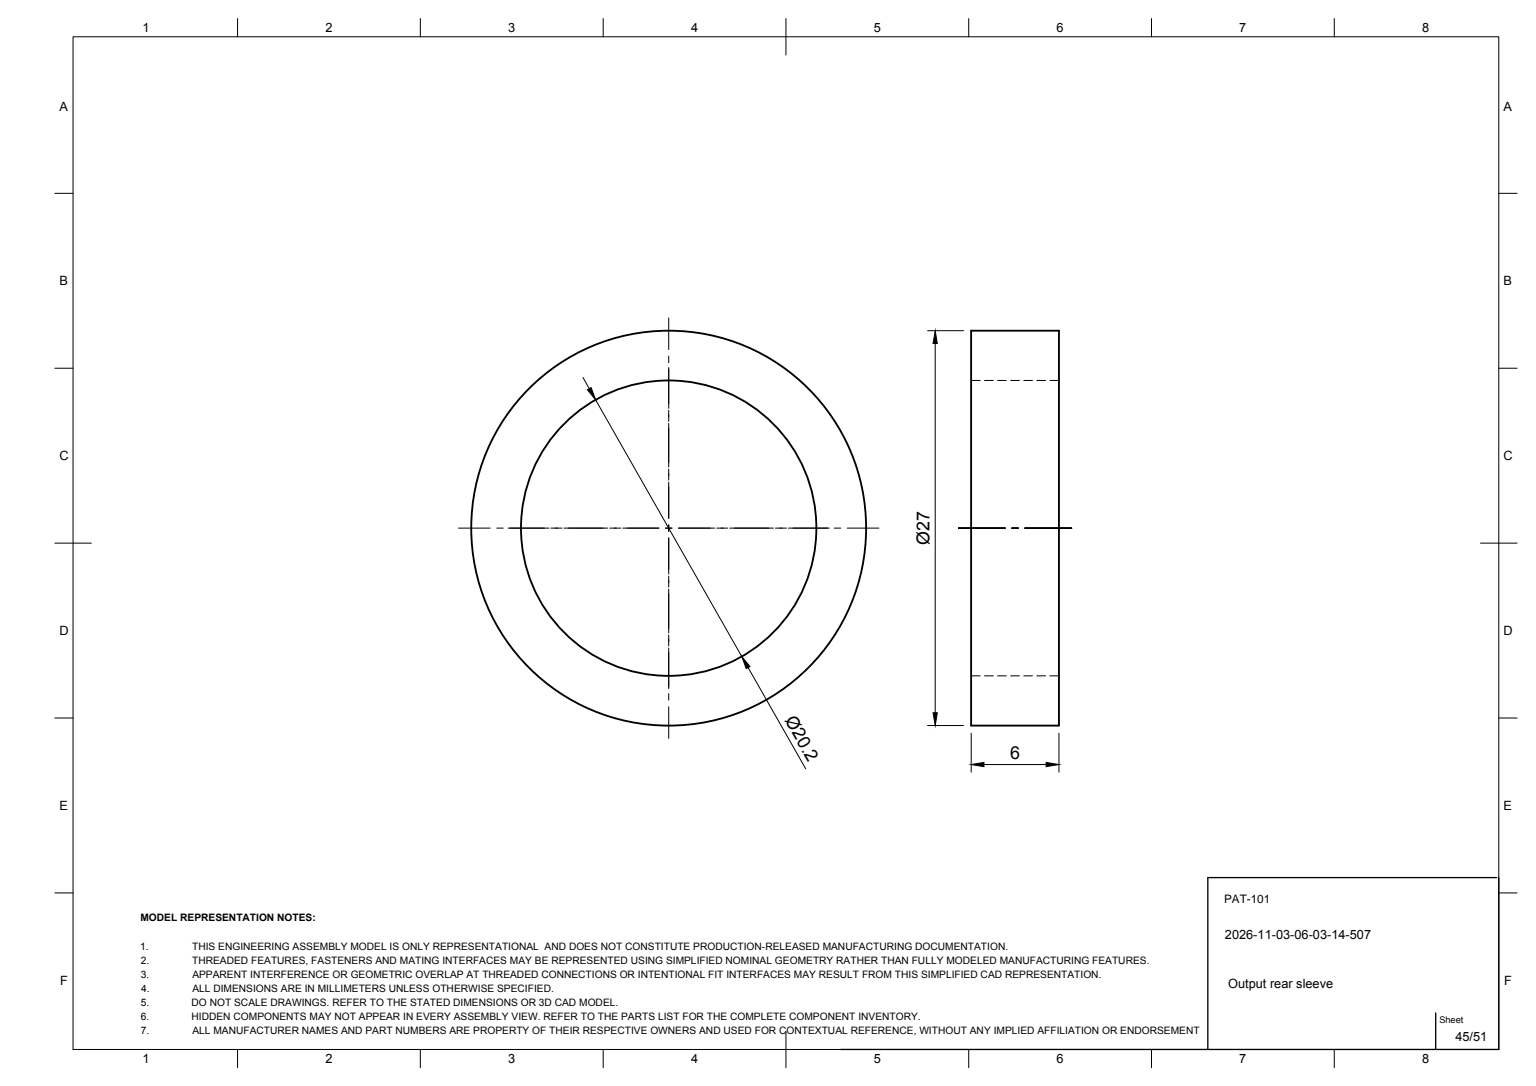
ISO-10303-21;
HEADER;
/* Generated by software containing ST-Developer
 * from STEP Tools, Inc. (www.steptools.com) 
 */

FILE_DESCRIPTION(
/* description */ ('Spur gear reduction stage 2-1 on bearing plates'),
/* implementation_level */ '2;1');

FILE_NAME(
/* name */ 'Output rear sleeve.step',
/* time_stamp */ '2026-10-28T03:22:07-07:00',
/* author */ (''),
/* organization */ (''),
/* preprocessor_version */ 'ST-DEVELOPER v20.2',
/* originating_system */ 'Autodesk Translation Framework v15.17.0.0',
/* authorisation */ '');

FILE_SCHEMA (('AUTOMOTIVE_DESIGN { 1 0 10303 214 3 1 1 }'));
ENDSEC;

DATA;
#10=MECHANICAL_DESIGN_GEOMETRIC_PRESENTATION_REPRESENTATION('',(#997),#53909);
#896=SHAPE_REPRESENTATION_RELATIONSHIP('SRR','None',#54127,#939);
#939=ADVANCED_BREP_SHAPE_REPRESENTATION('',(#1052),#53901);
#997=STYLED_ITEM('',(#54383),#1052);
#1052=MANIFOLD_SOLID_BREP('Body1',#11324);
#1220=FACE_BOUND('',#2746,.T.);
#1221=FACE_BOUND('',#2748,.T.);
#1424=PLANE('',#12706);
#1425=PLANE('',#12707);
#1935=FACE_OUTER_BOUND('',#2743,.T.);
#1936=FACE_OUTER_BOUND('',#2744,.T.);
#1937=FACE_OUTER_BOUND('',#2745,.T.);
#1938=FACE_OUTER_BOUND('',#2747,.T.);
#2743=EDGE_LOOP('',(#9232,#9233,#9234,#9235));
#2744=EDGE_LOOP('',(#9236,#9237,#9238,#9239));
#2745=EDGE_LOOP('',(#9240));
#2746=EDGE_LOOP('',(#9241));
#2747=EDGE_LOOP('',(#9242));
#2748=EDGE_LOOP('',(#9243));
#3386=LINE('',#29896,#4027);
#3387=LINE('',#29902,#4028);
#4027=VECTOR('',#15183,1.01);
#4028=VECTOR('',#15190,1.35);
#4670=CIRCLE('',#12701,1.01);
#4671=CIRCLE('',#12702,1.01);
#4672=CIRCLE('',#12704,1.35);
#4673=CIRCLE('',#12705,1.35);
#5422=VERTEX_POINT('',#29893);
#5423=VERTEX_POINT('',#29895);
#5424=VERTEX_POINT('',#29899);
#5425=VERTEX_POINT('',#29901);
#6758=EDGE_CURVE('',#5422,#5422,#4670,.T.);
#6759=EDGE_CURVE('',#5422,#5423,#3386,.T.);
#6760=EDGE_CURVE('',#5423,#5423,#4671,.T.);
#6761=EDGE_CURVE('',#5424,#5424,#4672,.T.);
#6762=EDGE_CURVE('',#5424,#5425,#3387,.T.);
#6763=EDGE_CURVE('',#5425,#5425,#4673,.T.);
#9232=ORIENTED_EDGE('',*,*,#6758,.F.);
#9233=ORIENTED_EDGE('',*,*,#6759,.T.);
#9234=ORIENTED_EDGE('',*,*,#6760,.T.);
#9235=ORIENTED_EDGE('',*,*,#6759,.F.);
#9236=ORIENTED_EDGE('',*,*,#6761,.F.);
#9237=ORIENTED_EDGE('',*,*,#6762,.T.);
#9238=ORIENTED_EDGE('',*,*,#6763,.T.);
#9239=ORIENTED_EDGE('',*,*,#6762,.F.);
#9240=ORIENTED_EDGE('',*,*,#6761,.T.);
#9241=ORIENTED_EDGE('',*,*,#6758,.T.);
#9242=ORIENTED_EDGE('',*,*,#6763,.F.);
#9243=ORIENTED_EDGE('',*,*,#6760,.F.);
#10568=CYLINDRICAL_SURFACE('',#12700,1.01);
#10569=CYLINDRICAL_SURFACE('',#12703,1.35);
#11055=ADVANCED_FACE('',(#1935),#10568,.F.);
#11056=ADVANCED_FACE('',(#1936),#10569,.T.);
#11057=ADVANCED_FACE('',(#1937,#1220),#1424,.T.);
#11058=ADVANCED_FACE('',(#1938,#1221),#1425,.F.);
#11324=CLOSED_SHELL('',(#11055,#11056,#11057,#11058));
#12699=AXIS2_PLACEMENT_3D('',#29891,#15177,#15178);
#12700=AXIS2_PLACEMENT_3D('',#29892,#15179,#15180);
#12701=AXIS2_PLACEMENT_3D('',#29894,#15181,#15182);
#12702=AXIS2_PLACEMENT_3D('',#29897,#15184,#15185);
#12703=AXIS2_PLACEMENT_3D('',#29898,#15186,#15187);
#12704=AXIS2_PLACEMENT_3D('',#29900,#15188,#15189);
#12705=AXIS2_PLACEMENT_3D('',#29903,#15191,#15192);
#12706=AXIS2_PLACEMENT_3D('',#29904,#15193,#15194);
#12707=AXIS2_PLACEMENT_3D('',#29905,#15195,#15196);
#15177=DIRECTION('axis',(0.,0.,1.));
#15178=DIRECTION('refdir',(1.,0.,0.));
#15179=DIRECTION('center_axis',(0.,1.,0.));
#15180=DIRECTION('ref_axis',(1.,0.,0.));
#15181=DIRECTION('center_axis',(0.,-1.,0.));
#15182=DIRECTION('ref_axis',(1.,0.,0.));
#15183=DIRECTION('',(0.,-1.,0.));
#15184=DIRECTION('center_axis',(0.,-1.,0.));
#15185=DIRECTION('ref_axis',(1.,0.,0.));
#15186=DIRECTION('center_axis',(0.,1.,0.));
#15187=DIRECTION('ref_axis',(1.,0.,0.));
#15188=DIRECTION('center_axis',(0.,1.,0.));
#15189=DIRECTION('ref_axis',(1.,0.,0.));
#15190=DIRECTION('',(0.,-1.,0.));
#15191=DIRECTION('center_axis',(0.,1.,0.));
#15192=DIRECTION('ref_axis',(1.,0.,0.));
#15193=DIRECTION('center_axis',(0.,1.,0.));
#15194=DIRECTION('ref_axis',(1.,0.,0.));
#15195=DIRECTION('center_axis',(0.,1.,0.));
#15196=DIRECTION('ref_axis',(1.,0.,0.));
#29891=CARTESIAN_POINT('',(0.,0.,0.));
#29892=CARTESIAN_POINT('Origin',(0.,2.2,0.));
#29893=CARTESIAN_POINT('',(-1.01,2.8,1.23689326713883E-16));
#29894=CARTESIAN_POINT('Origin',(0.,2.8,0.));
#29895=CARTESIAN_POINT('',(-1.01,2.2,1.23689326713883E-16));
#29896=CARTESIAN_POINT('',(-1.01,2.2,1.23689326713883E-16));
#29897=CARTESIAN_POINT('Origin',(0.,2.2,0.));
#29898=CARTESIAN_POINT('Origin',(0.,2.2,0.));
#29899=CARTESIAN_POINT('',(-1.35,2.8,1.65327317884893E-16));
#29900=CARTESIAN_POINT('Origin',(0.,2.8,0.));
#29901=CARTESIAN_POINT('',(-1.35,2.2,1.65327317884893E-16));
#29902=CARTESIAN_POINT('',(-1.35,2.2,1.65327317884893E-16));
#29903=CARTESIAN_POINT('Origin',(0.,2.2,0.));
#29904=CARTESIAN_POINT('Origin',(0.,2.8,0.));
#29905=CARTESIAN_POINT('Origin',(0.,2.2,0.));
#53851=UNCERTAINTY_MEASURE_WITH_UNIT(LENGTH_MEASURE(0.001),#53910,
'DISTANCE_ACCURACY_VALUE',
'Maximum model space distance between geometric entities at asserted c
onnectivities');
#53859=UNCERTAINTY_MEASURE_WITH_UNIT(LENGTH_MEASURE(0.001),#53910,
'DISTANCE_ACCURACY_VALUE',
'Maximum model space distance between geometric entities at asserted c
onnectivities');
#53901=(
GEOMETRIC_REPRESENTATION_CONTEXT(3)
GLOBAL_UNCERTAINTY_ASSIGNED_CONTEXT((#53851))
GLOBAL_UNIT_ASSIGNED_CONTEXT((#53910,#53912,#53913))
REPRESENTATION_CONTEXT('','3D')
);
#53909=(
GEOMETRIC_REPRESENTATION_CONTEXT(3)
GLOBAL_UNCERTAINTY_ASSIGNED_CONTEXT((#53859))
GLOBAL_UNIT_ASSIGNED_CONTEXT((#53910,#53912,#53913))
REPRESENTATION_CONTEXT('','3D')
);
#53910=(
LENGTH_UNIT()
NAMED_UNIT(*)
SI_UNIT(.CENTI.,.METRE.)
);
#53912=(
NAMED_UNIT(*)
PLANE_ANGLE_UNIT()
SI_UNIT($,.RADIAN.)
);
#53913=(
NAMED_UNIT(*)
SI_UNIT($,.STERADIAN.)
SOLID_ANGLE_UNIT()
);
#53955=SHAPE_DEFINITION_REPRESENTATION(#54053,#54127);
#54053=PRODUCT_DEFINITION_SHAPE('',$,#54177);
#54127=SHAPE_REPRESENTATION('',(#12699),#53901);
#54135=PRODUCT_DEFINITION_CONTEXT('part definition',#54284,'design');
#54177=PRODUCT_DEFINITION('Output rear sleeve','Output rear sleeve',#54226,
#54135);
#54226=PRODUCT_DEFINITION_FORMATION('',$,#54327);
#54284=APPLICATION_CONTEXT(
'Core Data for Automotive Mechanical Design Process');
#54285=PRODUCT_CONTEXT('part definition',#54284,'mechanical');
#54327=PRODUCT('Output rear sleeve','Output rear sleeve',
'Output rear sleeve',(#54285));
#54377=COLOUR_RGB('Light Blue',0.38,0.62,0.78);
#54378=FILL_AREA_STYLE_COLOUR('',#54377);
#54379=FILL_AREA_STYLE('',(#54378));
#54380=SURFACE_STYLE_FILL_AREA(#54379);
#54381=SURFACE_SIDE_STYLE('',(#54380));
#54382=SURFACE_STYLE_USAGE(.BOTH.,#54381);
#54383=PRESENTATION_STYLE_ASSIGNMENT((#54382));
ENDSEC;
END-ISO-10303-21;
